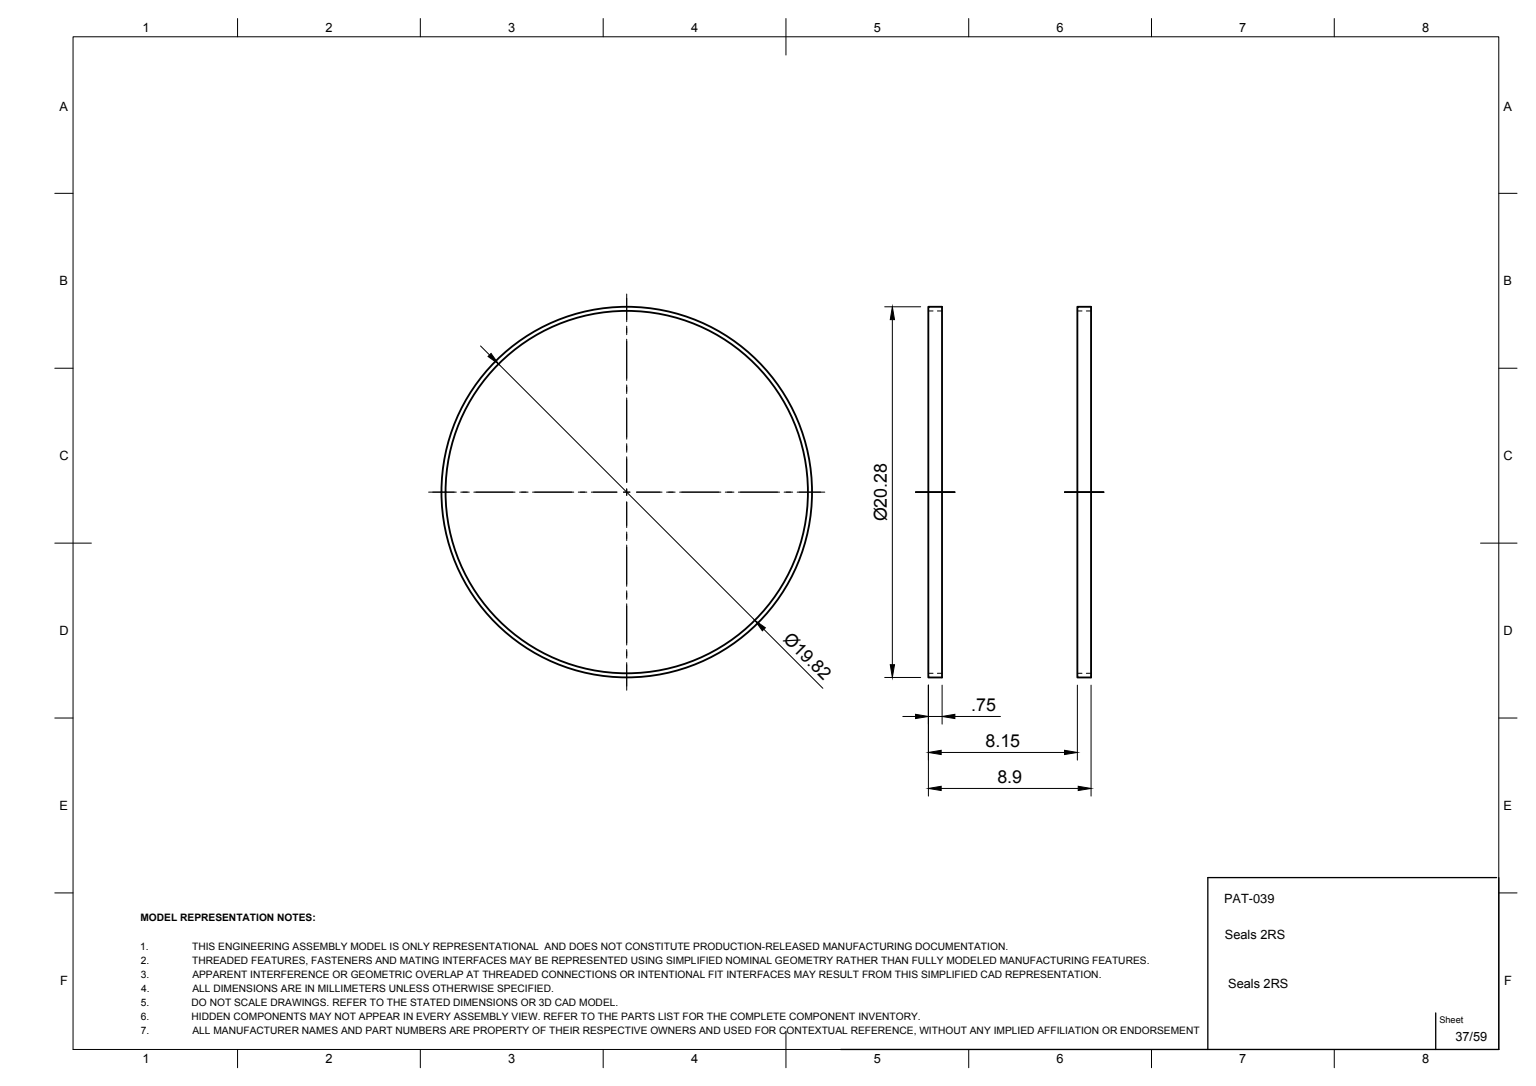
ISO-10303-21;
HEADER;
/* Generated by software containing ST-Developer
 * from STEP Tools, Inc. (www.steptools.com) 
 */

FILE_DESCRIPTION(
/* description */ ('Four-bar parallelogram arm'),
/* implementation_level */ '2;1');

FILE_NAME(
/* name */ 'Seals 2RS.step',
/* time_stamp */ '2026-10-28T03:24:55-07:00',
/* author */ (''),
/* organization */ (''),
/* preprocessor_version */ 'ST-DEVELOPER v20.2',
/* originating_system */ 'Autodesk Translation Framework v15.17.0.0',
/* authorisation */ '');

FILE_SCHEMA (('AUTOMOTIVE_DESIGN { 1 0 10303 214 3 1 1 }'));
ENDSEC;

DATA;
#10=MECHANICAL_DESIGN_GEOMETRIC_PRESENTATION_REPRESENTATION('',(#665,#666),#14512);
#558=SHAPE_REPRESENTATION_RELATIONSHIP('SRR','None',#14782,#608);
#608=ADVANCED_BREP_SHAPE_REPRESENTATION('',(#722,#723),#14497);
#665=STYLED_ITEM('',(#15087),#722);
#666=STYLED_ITEM('',(#15087),#723);
#722=MANIFOLD_SOLID_BREP('Body1',#7370);
#723=MANIFOLD_SOLID_BREP('Body2',#7371);
#942=FACE_BOUND('',#2131,.T.);
#943=FACE_BOUND('',#2134,.T.);
#944=FACE_BOUND('',#2137,.T.);
#945=FACE_BOUND('',#2140,.T.);
#1140=PLANE('',#8619);
#1141=PLANE('',#8624);
#1142=PLANE('',#8627);
#1143=PLANE('',#8632);
#1503=FACE_OUTER_BOUND('',#2130,.T.);
#1504=FACE_OUTER_BOUND('',#2132,.T.);
#1505=FACE_OUTER_BOUND('',#2133,.T.);
#1506=FACE_OUTER_BOUND('',#2135,.T.);
#1507=FACE_OUTER_BOUND('',#2136,.T.);
#1508=FACE_OUTER_BOUND('',#2138,.T.);
#1509=FACE_OUTER_BOUND('',#2139,.T.);
#1510=FACE_OUTER_BOUND('',#2141,.T.);
#2130=EDGE_LOOP('',(#6272));
#2131=EDGE_LOOP('',(#6273));
#2132=EDGE_LOOP('',(#6274,#6275,#6276,#6277));
#2133=EDGE_LOOP('',(#6278));
#2134=EDGE_LOOP('',(#6279));
#2135=EDGE_LOOP('',(#6280,#6281,#6282,#6283));
#2136=EDGE_LOOP('',(#6284));
#2137=EDGE_LOOP('',(#6285));
#2138=EDGE_LOOP('',(#6286,#6287,#6288,#6289));
#2139=EDGE_LOOP('',(#6290));
#2140=EDGE_LOOP('',(#6291));
#2141=EDGE_LOOP('',(#6292,#6293,#6294,#6295));
#2592=LINE('',#13797,#2986);
#2593=LINE('',#13802,#2987);
#2594=LINE('',#13811,#2988);
#2595=LINE('',#13816,#2989);
#2986=VECTOR('',#10622,1.013815);
#2987=VECTOR('',#10629,0.991185);
#2988=VECTOR('',#10640,1.013815);
#2989=VECTOR('',#10647,0.991185);
#3438=CIRCLE('',#8620,1.013815);
#3439=CIRCLE('',#8621,0.991185);
#3440=CIRCLE('',#8623,1.013815);
#3441=CIRCLE('',#8625,0.991185);
#3442=CIRCLE('',#8628,1.013815);
#3443=CIRCLE('',#8629,0.991185);
#3444=CIRCLE('',#8631,1.013815);
#3445=CIRCLE('',#8633,0.991185);
#3980=VERTEX_POINT('',#13790);
#3981=VERTEX_POINT('',#13792);
#3982=VERTEX_POINT('',#13795);
#3983=VERTEX_POINT('',#13799);
#3984=VERTEX_POINT('',#13804);
#3985=VERTEX_POINT('',#13806);
#3986=VERTEX_POINT('',#13809);
#3987=VERTEX_POINT('',#13813);
#4767=EDGE_CURVE('',#3980,#3980,#3438,.T.);
#4768=EDGE_CURVE('',#3981,#3981,#3439,.T.);
#4769=EDGE_CURVE('',#3982,#3982,#3440,.T.);
#4770=EDGE_CURVE('',#3982,#3980,#2592,.T.);
#4771=EDGE_CURVE('',#3983,#3983,#3441,.T.);
#4772=EDGE_CURVE('',#3983,#3981,#2593,.T.);
#4773=EDGE_CURVE('',#3984,#3984,#3442,.T.);
#4774=EDGE_CURVE('',#3985,#3985,#3443,.T.);
#4775=EDGE_CURVE('',#3986,#3986,#3444,.T.);
#4776=EDGE_CURVE('',#3986,#3984,#2594,.T.);
#4777=EDGE_CURVE('',#3987,#3987,#3445,.T.);
#4778=EDGE_CURVE('',#3987,#3985,#2595,.T.);
#6272=ORIENTED_EDGE('',*,*,#4767,.F.);
#6273=ORIENTED_EDGE('',*,*,#4768,.T.);
#6274=ORIENTED_EDGE('',*,*,#4769,.F.);
#6275=ORIENTED_EDGE('',*,*,#4770,.T.);
#6276=ORIENTED_EDGE('',*,*,#4767,.T.);
#6277=ORIENTED_EDGE('',*,*,#4770,.F.);
#6278=ORIENTED_EDGE('',*,*,#4769,.T.);
#6279=ORIENTED_EDGE('',*,*,#4771,.F.);
#6280=ORIENTED_EDGE('',*,*,#4771,.T.);
#6281=ORIENTED_EDGE('',*,*,#4772,.T.);
#6282=ORIENTED_EDGE('',*,*,#4768,.F.);
#6283=ORIENTED_EDGE('',*,*,#4772,.F.);
#6284=ORIENTED_EDGE('',*,*,#4773,.F.);
#6285=ORIENTED_EDGE('',*,*,#4774,.T.);
#6286=ORIENTED_EDGE('',*,*,#4775,.F.);
#6287=ORIENTED_EDGE('',*,*,#4776,.T.);
#6288=ORIENTED_EDGE('',*,*,#4773,.T.);
#6289=ORIENTED_EDGE('',*,*,#4776,.F.);
#6290=ORIENTED_EDGE('',*,*,#4775,.T.);
#6291=ORIENTED_EDGE('',*,*,#4777,.F.);
#6292=ORIENTED_EDGE('',*,*,#4777,.T.);
#6293=ORIENTED_EDGE('',*,*,#4778,.T.);
#6294=ORIENTED_EDGE('',*,*,#4774,.F.);
#6295=ORIENTED_EDGE('',*,*,#4778,.F.);
#6856=CYLINDRICAL_SURFACE('',#8622,1.013815);
#6857=CYLINDRICAL_SURFACE('',#8626,0.991185);
#6858=CYLINDRICAL_SURFACE('',#8630,1.013815);
#6859=CYLINDRICAL_SURFACE('',#8634,0.991185);
#7208=ADVANCED_FACE('',(#1503,#942),#1140,.T.);
#7209=ADVANCED_FACE('',(#1504),#6856,.T.);
#7210=ADVANCED_FACE('',(#1505,#943),#1141,.T.);
#7211=ADVANCED_FACE('',(#1506),#6857,.F.);
#7212=ADVANCED_FACE('',(#1507,#944),#1142,.T.);
#7213=ADVANCED_FACE('',(#1508),#6858,.T.);
#7214=ADVANCED_FACE('',(#1509,#945),#1143,.T.);
#7215=ADVANCED_FACE('',(#1510),#6859,.F.);
#7370=CLOSED_SHELL('',(#7208,#7209,#7210,#7211));
#7371=CLOSED_SHELL('',(#7212,#7213,#7214,#7215));
#8618=AXIS2_PLACEMENT_3D('',#13788,#10610,#10611);
#8619=AXIS2_PLACEMENT_3D('',#13789,#10612,#10613);
#8620=AXIS2_PLACEMENT_3D('',#13791,#10614,#10615);
#8621=AXIS2_PLACEMENT_3D('',#13793,#10616,#10617);
#8622=AXIS2_PLACEMENT_3D('',#13794,#10618,#10619);
#8623=AXIS2_PLACEMENT_3D('',#13796,#10620,#10621);
#8624=AXIS2_PLACEMENT_3D('',#13798,#10623,#10624);
#8625=AXIS2_PLACEMENT_3D('',#13800,#10625,#10626);
#8626=AXIS2_PLACEMENT_3D('',#13801,#10627,#10628);
#8627=AXIS2_PLACEMENT_3D('',#13803,#10630,#10631);
#8628=AXIS2_PLACEMENT_3D('',#13805,#10632,#10633);
#8629=AXIS2_PLACEMENT_3D('',#13807,#10634,#10635);
#8630=AXIS2_PLACEMENT_3D('',#13808,#10636,#10637);
#8631=AXIS2_PLACEMENT_3D('',#13810,#10638,#10639);
#8632=AXIS2_PLACEMENT_3D('',#13812,#10641,#10642);
#8633=AXIS2_PLACEMENT_3D('',#13814,#10643,#10644);
#8634=AXIS2_PLACEMENT_3D('',#13815,#10645,#10646);
#10610=DIRECTION('axis',(0.,0.,1.));
#10611=DIRECTION('refdir',(1.,0.,0.));
#10612=DIRECTION('center_axis',(0.,1.,0.));
#10613=DIRECTION('ref_axis',(0.,0.,1.));
#10614=DIRECTION('center_axis',(0.,-1.,0.));
#10615=DIRECTION('ref_axis',(1.,0.,0.));
#10616=DIRECTION('center_axis',(0.,-1.,0.));
#10617=DIRECTION('ref_axis',(1.,0.,0.));
#10618=DIRECTION('center_axis',(0.,-1.,0.));
#10619=DIRECTION('ref_axis',(1.,0.,0.));
#10620=DIRECTION('center_axis',(0.,-1.,0.));
#10621=DIRECTION('ref_axis',(1.,0.,0.));
#10622=DIRECTION('',(0.,1.,0.));
#10623=DIRECTION('center_axis',(0.,-1.,0.));
#10624=DIRECTION('ref_axis',(0.,0.,-1.));
#10625=DIRECTION('center_axis',(0.,-1.,0.));
#10626=DIRECTION('ref_axis',(1.,0.,0.));
#10627=DIRECTION('center_axis',(0.,-1.,0.));
#10628=DIRECTION('ref_axis',(1.,0.,0.));
#10629=DIRECTION('',(0.,1.,0.));
#10630=DIRECTION('center_axis',(0.,1.,0.));
#10631=DIRECTION('ref_axis',(0.,0.,1.));
#10632=DIRECTION('center_axis',(0.,-1.,0.));
#10633=DIRECTION('ref_axis',(1.,0.,0.));
#10634=DIRECTION('center_axis',(0.,-1.,0.));
#10635=DIRECTION('ref_axis',(1.,0.,0.));
#10636=DIRECTION('center_axis',(0.,-1.,0.));
#10637=DIRECTION('ref_axis',(1.,0.,0.));
#10638=DIRECTION('center_axis',(0.,-1.,0.));
#10639=DIRECTION('ref_axis',(1.,0.,0.));
#10640=DIRECTION('',(0.,1.,0.));
#10641=DIRECTION('center_axis',(0.,-1.,0.));
#10642=DIRECTION('ref_axis',(0.,0.,-1.));
#10643=DIRECTION('center_axis',(0.,-1.,0.));
#10644=DIRECTION('ref_axis',(1.,0.,0.));
#10645=DIRECTION('center_axis',(0.,-1.,0.));
#10646=DIRECTION('ref_axis',(1.,0.,0.));
#10647=DIRECTION('',(0.,1.,0.));
#13788=CARTESIAN_POINT('',(0.,0.,0.));
#13789=CARTESIAN_POINT('Origin',(1.013815,0.445,0.));
#13790=CARTESIAN_POINT('',(-1.013815,0.445,-1.24156529467757E-16));
#13791=CARTESIAN_POINT('Origin',(0.,0.445,0.));
#13792=CARTESIAN_POINT('',(-0.991185,0.445,-1.21385153761287E-16));
#13793=CARTESIAN_POINT('Origin',(0.,0.445,0.));
#13794=CARTESIAN_POINT('Origin',(0.,0.4075,0.));
#13795=CARTESIAN_POINT('',(-1.013815,0.37,-1.24156529467757E-16));
#13796=CARTESIAN_POINT('Origin',(0.,0.37,0.));
#13797=CARTESIAN_POINT('',(-1.013815,0.4075,-1.24156529467757E-16));
#13798=CARTESIAN_POINT('Origin',(0.991185,0.37,0.));
#13799=CARTESIAN_POINT('',(-0.991185,0.37,-1.21385153761287E-16));
#13800=CARTESIAN_POINT('Origin',(0.,0.37,0.));
#13801=CARTESIAN_POINT('Origin',(0.,0.4075,0.));
#13802=CARTESIAN_POINT('',(-0.991185,0.4075,-1.21385153761287E-16));
#13803=CARTESIAN_POINT('Origin',(1.013815,-0.37,0.));
#13804=CARTESIAN_POINT('',(-1.013815,-0.37,-1.24156529467757E-16));
#13805=CARTESIAN_POINT('Origin',(0.,-0.37,0.));
#13806=CARTESIAN_POINT('',(-0.991185,-0.37,-1.21385153761287E-16));
#13807=CARTESIAN_POINT('Origin',(0.,-0.37,0.));
#13808=CARTESIAN_POINT('Origin',(0.,-0.4075,0.));
#13809=CARTESIAN_POINT('',(-1.013815,-0.445,-1.24156529467757E-16));
#13810=CARTESIAN_POINT('Origin',(0.,-0.445,0.));
#13811=CARTESIAN_POINT('',(-1.013815,-0.4075,-1.24156529467757E-16));
#13812=CARTESIAN_POINT('Origin',(0.991185,-0.445,0.));
#13813=CARTESIAN_POINT('',(-0.991185,-0.445,-1.21385153761287E-16));
#13814=CARTESIAN_POINT('Origin',(0.,-0.445,0.));
#13815=CARTESIAN_POINT('Origin',(0.,-0.4075,0.));
#13816=CARTESIAN_POINT('',(-0.991185,-0.4075,-1.21385153761287E-16));
#14440=UNCERTAINTY_MEASURE_WITH_UNIT(LENGTH_MEASURE(0.001),#14513,
'DISTANCE_ACCURACY_VALUE',
'Maximum model space distance between geometric entities at asserted c
onnectivities');
#14455=UNCERTAINTY_MEASURE_WITH_UNIT(LENGTH_MEASURE(0.001),#14513,
'DISTANCE_ACCURACY_VALUE',
'Maximum model space distance between geometric entities at asserted c
onnectivities');
#14497=(
GEOMETRIC_REPRESENTATION_CONTEXT(3)
GLOBAL_UNCERTAINTY_ASSIGNED_CONTEXT((#14440))
GLOBAL_UNIT_ASSIGNED_CONTEXT((#14513,#14515,#14516))
REPRESENTATION_CONTEXT('','3D')
);
#14512=(
GEOMETRIC_REPRESENTATION_CONTEXT(3)
GLOBAL_UNCERTAINTY_ASSIGNED_CONTEXT((#14455))
GLOBAL_UNIT_ASSIGNED_CONTEXT((#14513,#14515,#14516))
REPRESENTATION_CONTEXT('','3D')
);
#14513=(
LENGTH_UNIT()
NAMED_UNIT(*)
SI_UNIT(.CENTI.,.METRE.)
);
#14515=(
NAMED_UNIT(*)
PLANE_ANGLE_UNIT()
SI_UNIT($,.RADIAN.)
);
#14516=(
NAMED_UNIT(*)
SI_UNIT($,.STERADIAN.)
SOLID_ANGLE_UNIT()
);
#14558=SHAPE_DEFINITION_REPRESENTATION(#14614,#14782);
#14614=PRODUCT_DEFINITION_SHAPE('',$,#14839);
#14782=SHAPE_REPRESENTATION('',(#8618),#14497);
#14797=PRODUCT_DEFINITION_CONTEXT('part definition',#14967,'design');
#14839=PRODUCT_DEFINITION('Seals 2RS','Seals 2RS',#14895,#14797);
#14895=PRODUCT_DEFINITION_FORMATION('',$,#15010);
#14967=APPLICATION_CONTEXT(
'Core Data for Automotive Mechanical Design Process');
#14968=PRODUCT_CONTEXT('part definition',#14967,'mechanical');
#15010=PRODUCT('Seals 2RS','Seals 2RS','Seals 2RS',(#14968));
#15081=COLOUR_RGB('Grey',0.48,0.52,0.57);
#15082=FILL_AREA_STYLE_COLOUR('',#15081);
#15083=FILL_AREA_STYLE('',(#15082));
#15084=SURFACE_STYLE_FILL_AREA(#15083);
#15085=SURFACE_SIDE_STYLE('',(#15084));
#15086=SURFACE_STYLE_USAGE(.BOTH.,#15085);
#15087=PRESENTATION_STYLE_ASSIGNMENT((#15086));
ENDSEC;
END-ISO-10303-21;
